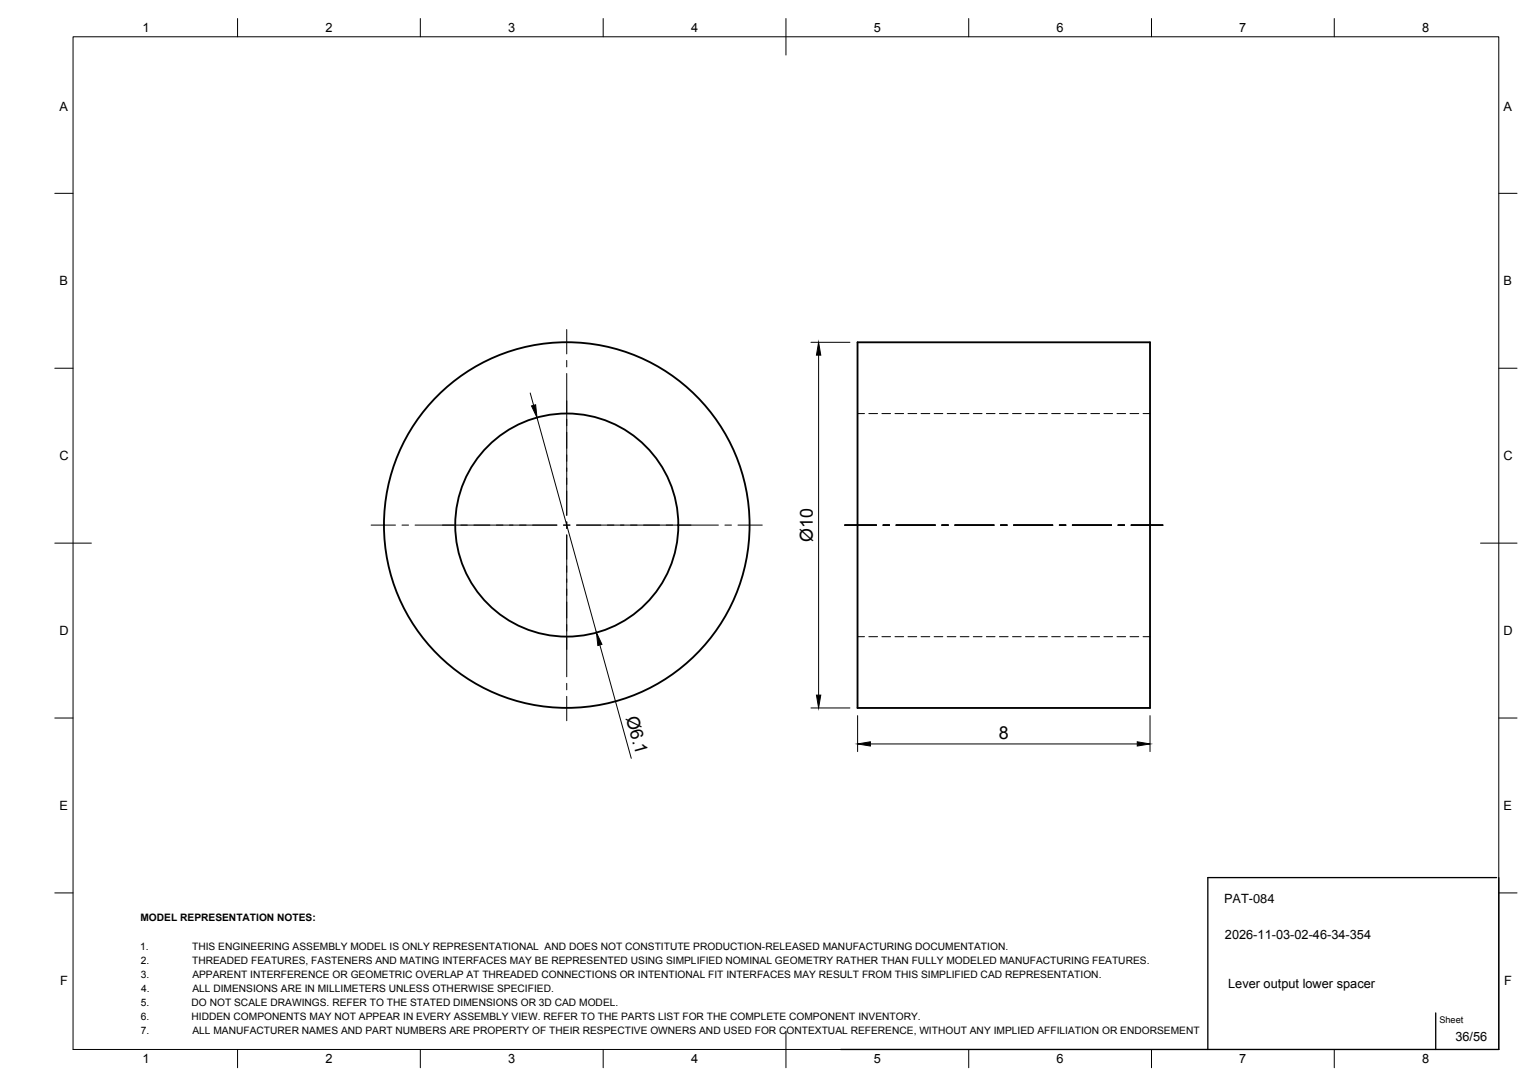
ISO-10303-21;
HEADER;
/* Generated by software containing ST-Developer
 * from STEP Tools, Inc. (www.steptools.com) 
 */

FILE_DESCRIPTION(
/* description */ ('Quick-return (Whitworth) mechanism'),
/* implementation_level */ '2;1');

FILE_NAME(
/* name */ 'Lever output lower spacer.step',
/* time_stamp */ '2026-10-28T03:25:57-07:00',
/* author */ (''),
/* organization */ (''),
/* preprocessor_version */ 'ST-DEVELOPER v20.2',
/* originating_system */ 'Autodesk Translation Framework v15.17.0.0',
/* authorisation */ '');

FILE_SCHEMA (('AUTOMOTIVE_DESIGN { 1 0 10303 214 3 1 1 }'));
ENDSEC;

DATA;
#10=MECHANICAL_DESIGN_GEOMETRIC_PRESENTATION_REPRESENTATION('',(#524),#14878);
#428=SHAPE_REPRESENTATION_RELATIONSHIP('SRR','None',#15099,#472);
#472=ADVANCED_BREP_SHAPE_REPRESENTATION('',(#575),#14856);
#524=STYLED_ITEM('',(#15399),#575);
#575=MANIFOLD_SOLID_BREP('Body1',#7879);
#740=FACE_BOUND('',#1971,.T.);
#741=FACE_BOUND('',#1973,.T.);
#933=PLANE('',#9055);
#934=PLANE('',#9056);
#1353=FACE_OUTER_BOUND('',#1968,.T.);
#1354=FACE_OUTER_BOUND('',#1969,.T.);
#1355=FACE_OUTER_BOUND('',#1970,.T.);
#1356=FACE_OUTER_BOUND('',#1972,.T.);
#1968=EDGE_LOOP('',(#6516,#6517,#6518,#6519));
#1969=EDGE_LOOP('',(#6520,#6521,#6522,#6523));
#1970=EDGE_LOOP('',(#6524));
#1971=EDGE_LOOP('',(#6525));
#1972=EDGE_LOOP('',(#6526));
#1973=EDGE_LOOP('',(#6527));
#2439=LINE('',#13944,#2962);
#2440=LINE('',#13950,#2963);
#2962=VECTOR('',#11000,0.305);
#2963=VECTOR('',#11007,0.5);
#3538=CIRCLE('',#9050,0.305);
#3539=CIRCLE('',#9051,0.305);
#3540=CIRCLE('',#9053,0.5);
#3541=CIRCLE('',#9054,0.5);
#4059=VERTEX_POINT('',#13941);
#4060=VERTEX_POINT('',#13943);
#4061=VERTEX_POINT('',#13947);
#4062=VERTEX_POINT('',#13949);
#4915=EDGE_CURVE('',#4059,#4059,#3538,.T.);
#4916=EDGE_CURVE('',#4059,#4060,#2439,.T.);
#4917=EDGE_CURVE('',#4060,#4060,#3539,.T.);
#4918=EDGE_CURVE('',#4061,#4061,#3540,.T.);
#4919=EDGE_CURVE('',#4061,#4062,#2440,.T.);
#4920=EDGE_CURVE('',#4062,#4062,#3541,.T.);
#6516=ORIENTED_EDGE('',*,*,#4915,.F.);
#6517=ORIENTED_EDGE('',*,*,#4916,.T.);
#6518=ORIENTED_EDGE('',*,*,#4917,.T.);
#6519=ORIENTED_EDGE('',*,*,#4916,.F.);
#6520=ORIENTED_EDGE('',*,*,#4918,.F.);
#6521=ORIENTED_EDGE('',*,*,#4919,.T.);
#6522=ORIENTED_EDGE('',*,*,#4920,.T.);
#6523=ORIENTED_EDGE('',*,*,#4919,.F.);
#6524=ORIENTED_EDGE('',*,*,#4918,.T.);
#6525=ORIENTED_EDGE('',*,*,#4915,.T.);
#6526=ORIENTED_EDGE('',*,*,#4920,.F.);
#6527=ORIENTED_EDGE('',*,*,#4917,.F.);
#7339=CYLINDRICAL_SURFACE('',#9049,0.305);
#7340=CYLINDRICAL_SURFACE('',#9052,0.5);
#7684=ADVANCED_FACE('',(#1353),#7339,.F.);
#7685=ADVANCED_FACE('',(#1354),#7340,.T.);
#7686=ADVANCED_FACE('',(#1355,#740),#933,.T.);
#7687=ADVANCED_FACE('',(#1356,#741),#934,.F.);
#7879=CLOSED_SHELL('',(#7684,#7685,#7686,#7687));
#9048=AXIS2_PLACEMENT_3D('',#13939,#10994,#10995);
#9049=AXIS2_PLACEMENT_3D('',#13940,#10996,#10997);
#9050=AXIS2_PLACEMENT_3D('',#13942,#10998,#10999);
#9051=AXIS2_PLACEMENT_3D('',#13945,#11001,#11002);
#9052=AXIS2_PLACEMENT_3D('',#13946,#11003,#11004);
#9053=AXIS2_PLACEMENT_3D('',#13948,#11005,#11006);
#9054=AXIS2_PLACEMENT_3D('',#13951,#11008,#11009);
#9055=AXIS2_PLACEMENT_3D('',#13952,#11010,#11011);
#9056=AXIS2_PLACEMENT_3D('',#13953,#11012,#11013);
#10994=DIRECTION('axis',(0.,0.,1.));
#10995=DIRECTION('refdir',(1.,0.,0.));
#10996=DIRECTION('center_axis',(0.,0.,1.));
#10997=DIRECTION('ref_axis',(1.,0.,0.));
#10998=DIRECTION('center_axis',(0.,0.,-1.));
#10999=DIRECTION('ref_axis',(1.,0.,0.));
#11000=DIRECTION('',(0.,0.,-1.));
#11001=DIRECTION('center_axis',(0.,0.,-1.));
#11002=DIRECTION('ref_axis',(1.,0.,0.));
#11003=DIRECTION('center_axis',(0.,0.,1.));
#11004=DIRECTION('ref_axis',(1.,0.,0.));
#11005=DIRECTION('center_axis',(0.,0.,1.));
#11006=DIRECTION('ref_axis',(1.,0.,0.));
#11007=DIRECTION('',(0.,0.,-1.));
#11008=DIRECTION('center_axis',(0.,0.,1.));
#11009=DIRECTION('ref_axis',(1.,0.,0.));
#11010=DIRECTION('center_axis',(0.,0.,1.));
#11011=DIRECTION('ref_axis',(1.,0.,0.));
#11012=DIRECTION('center_axis',(0.,0.,1.));
#11013=DIRECTION('ref_axis',(1.,0.,0.));
#13939=CARTESIAN_POINT('',(0.,0.,0.));
#13940=CARTESIAN_POINT('Origin',(0.,12.,7.6));
#13941=CARTESIAN_POINT('',(-0.305,12.,8.4));
#13942=CARTESIAN_POINT('Origin',(0.,12.,8.4));
#13943=CARTESIAN_POINT('',(-0.305,12.,7.6));
#13944=CARTESIAN_POINT('',(-0.305,12.,7.6));
#13945=CARTESIAN_POINT('Origin',(0.,12.,7.6));
#13946=CARTESIAN_POINT('Origin',(0.,12.,7.6));
#13947=CARTESIAN_POINT('',(-0.5,12.,8.4));
#13948=CARTESIAN_POINT('Origin',(0.,12.,8.4));
#13949=CARTESIAN_POINT('',(-0.5,12.,7.6));
#13950=CARTESIAN_POINT('',(-0.5,12.,7.6));
#13951=CARTESIAN_POINT('Origin',(0.,12.,7.6));
#13952=CARTESIAN_POINT('Origin',(0.,12.,8.4));
#13953=CARTESIAN_POINT('Origin',(0.,12.,7.6));
#14802=UNCERTAINTY_MEASURE_WITH_UNIT(LENGTH_MEASURE(0.001),#14879,
'DISTANCE_ACCURACY_VALUE',
'Maximum model space distance between geometric entities at asserted c
onnectivities');
#14824=UNCERTAINTY_MEASURE_WITH_UNIT(LENGTH_MEASURE(0.001),#14879,
'DISTANCE_ACCURACY_VALUE',
'Maximum model space distance between geometric entities at asserted c
onnectivities');
#14856=(
GEOMETRIC_REPRESENTATION_CONTEXT(3)
GLOBAL_UNCERTAINTY_ASSIGNED_CONTEXT((#14802))
GLOBAL_UNIT_ASSIGNED_CONTEXT((#14879,#14881,#14882))
REPRESENTATION_CONTEXT('','3D')
);
#14878=(
GEOMETRIC_REPRESENTATION_CONTEXT(3)
GLOBAL_UNCERTAINTY_ASSIGNED_CONTEXT((#14824))
GLOBAL_UNIT_ASSIGNED_CONTEXT((#14879,#14881,#14882))
REPRESENTATION_CONTEXT('','3D')
);
#14879=(
LENGTH_UNIT()
NAMED_UNIT(*)
SI_UNIT(.CENTI.,.METRE.)
);
#14881=(
NAMED_UNIT(*)
PLANE_ANGLE_UNIT()
SI_UNIT($,.RADIAN.)
);
#14882=(
NAMED_UNIT(*)
SI_UNIT($,.STERADIAN.)
SOLID_ANGLE_UNIT()
);
#14914=SHAPE_DEFINITION_REPRESENTATION(#14972,#15099);
#14972=PRODUCT_DEFINITION_SHAPE('',$,#15153);
#15099=SHAPE_REPRESENTATION('',(#9048),#14856);
#15121=PRODUCT_DEFINITION_CONTEXT('part definition',#15282,'design');
#15153=PRODUCT_DEFINITION('Lever output lower spacer',
'Lever output lower spacer',#15206,#15121);
#15206=PRODUCT_DEFINITION_FORMATION('',$,#15315);
#15282=APPLICATION_CONTEXT(
'Core Data for Automotive Mechanical Design Process');
#15283=PRODUCT_CONTEXT('part definition',#15282,'mechanical');
#15315=PRODUCT('Lever output lower spacer','Lever output lower spacer',
'Lever output lower spacer',(#15283));
#15393=COLOUR_RGB('Sky Blue',0.24,0.69,0.87);
#15394=FILL_AREA_STYLE_COLOUR('',#15393);
#15395=FILL_AREA_STYLE('',(#15394));
#15396=SURFACE_STYLE_FILL_AREA(#15395);
#15397=SURFACE_SIDE_STYLE('',(#15396));
#15398=SURFACE_STYLE_USAGE(.BOTH.,#15397);
#15399=PRESENTATION_STYLE_ASSIGNMENT((#15398));
ENDSEC;
END-ISO-10303-21;
